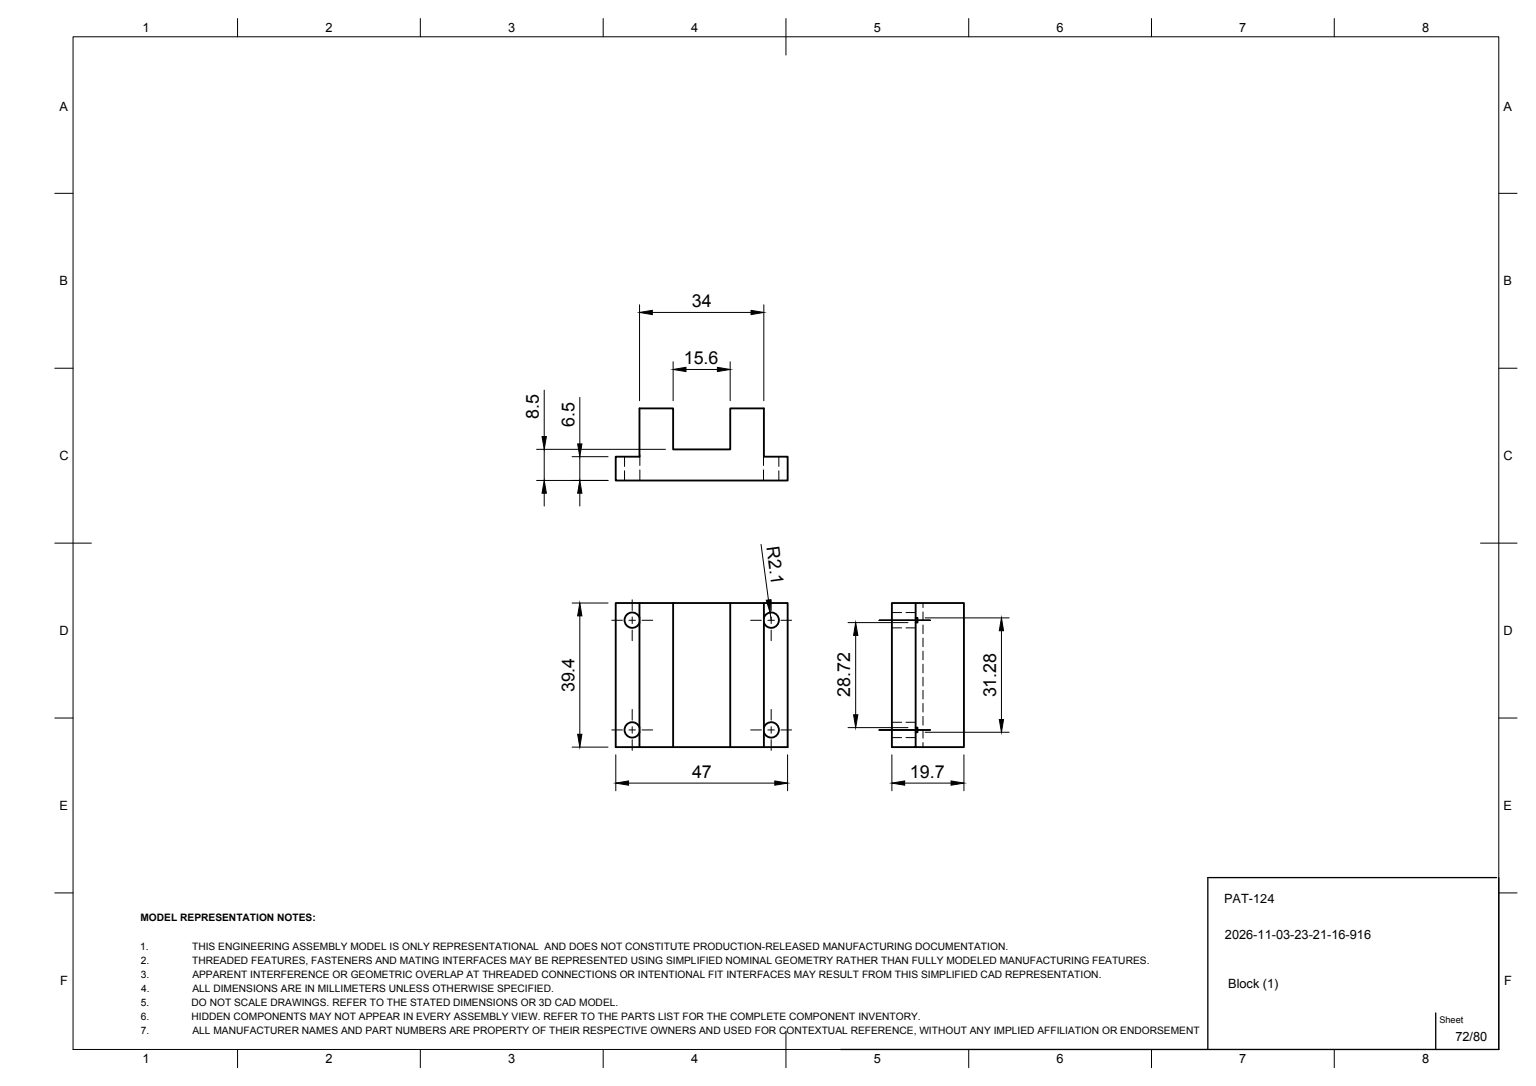
ISO-10303-21;
HEADER;
/* Generated by software containing ST-Developer
 * from STEP Tools, Inc. (www.steptools.com) 
 */

FILE_DESCRIPTION(
/* description */ ('XY cross-slide table'),
/* implementation_level */ '2;1');

FILE_NAME(
/* name */ 'Block (1).step',
/* time_stamp */ '2026-10-28T03:22:46-07:00',
/* author */ (''),
/* organization */ (''),
/* preprocessor_version */ 'ST-DEVELOPER v20.2',
/* originating_system */ 'Autodesk Translation Framework v15.17.0.0',
/* authorisation */ '');

FILE_SCHEMA (('AUTOMOTIVE_DESIGN { 1 0 10303 214 3 1 1 }'));
ENDSEC;

DATA;
#10=MECHANICAL_DESIGN_GEOMETRIC_PRESENTATION_REPRESENTATION('',(#1765),#62984);
#1569=SHAPE_REPRESENTATION_RELATIONSHIP('SRR','None',#63428,#1652);
#1652=ADVANCED_BREP_SHAPE_REPRESENTATION('',(#1873),#62965);
#1765=STYLED_ITEM('',(#63891),#1873);
#1873=MANIFOLD_SOLID_BREP('Body1',#23064);
#2253=FACE_BOUND('',#5529,.T.);
#2254=FACE_BOUND('',#5530,.T.);
#2255=FACE_BOUND('',#5531,.T.);
#2256=FACE_BOUND('',#5532,.T.);
#2731=PLANE('',#25907);
#2732=PLANE('',#25913);
#2733=PLANE('',#25919);
#2734=PLANE('',#25925);
#2735=PLANE('',#25931);
#2736=PLANE('',#25932);
#2737=PLANE('',#25933);
#2738=PLANE('',#25934);
#2739=PLANE('',#25935);
#2740=PLANE('',#25936);
#2741=PLANE('',#25937);
#2742=PLANE('',#25938);
#2743=PLANE('',#25939);
#2744=PLANE('',#25940);
#2745=PLANE('',#25941);
#2746=PLANE('',#25942);
#2747=PLANE('',#25943);
#2748=PLANE('',#25944);
#3835=FACE_OUTER_BOUND('',#5515,.T.);
#3836=FACE_OUTER_BOUND('',#5516,.T.);
#3837=FACE_OUTER_BOUND('',#5517,.T.);
#3838=FACE_OUTER_BOUND('',#5518,.T.);
#3839=FACE_OUTER_BOUND('',#5519,.T.);
#3840=FACE_OUTER_BOUND('',#5520,.T.);
#3841=FACE_OUTER_BOUND('',#5521,.T.);
#3842=FACE_OUTER_BOUND('',#5522,.T.);
#3843=FACE_OUTER_BOUND('',#5523,.T.);
#3844=FACE_OUTER_BOUND('',#5524,.T.);
#3845=FACE_OUTER_BOUND('',#5525,.T.);
#3846=FACE_OUTER_BOUND('',#5526,.T.);
#3847=FACE_OUTER_BOUND('',#5527,.T.);
#3848=FACE_OUTER_BOUND('',#5528,.T.);
#3849=FACE_OUTER_BOUND('',#5533,.T.);
#3850=FACE_OUTER_BOUND('',#5534,.T.);
#3851=FACE_OUTER_BOUND('',#5535,.T.);
#3852=FACE_OUTER_BOUND('',#5536,.T.);
#3853=FACE_OUTER_BOUND('',#5537,.T.);
#3854=FACE_OUTER_BOUND('',#5538,.T.);
#3855=FACE_OUTER_BOUND('',#5539,.T.);
#3856=FACE_OUTER_BOUND('',#5540,.T.);
#5515=EDGE_LOOP('',(#19290,#19291));
#5516=EDGE_LOOP('',(#19292,#19293,#19294,#19295,#19296,#19297,#19298,#19299));
#5517=EDGE_LOOP('',(#19300,#19301));
#5518=EDGE_LOOP('',(#19302,#19303,#19304,#19305,#19306,#19307,#19308,#19309));
#5519=EDGE_LOOP('',(#19310,#19311));
#5520=EDGE_LOOP('',(#19312,#19313,#19314,#19315,#19316,#19317,#19318,#19319));
#5521=EDGE_LOOP('',(#19320,#19321));
#5522=EDGE_LOOP('',(#19322,#19323,#19324,#19325,#19326,#19327,#19328,#19329));
#5523=EDGE_LOOP('',(#19330,#19331,#19332,#19333,#19334,#19335,#19336,#19337,
#19338,#19339,#19340,#19341));
#5524=EDGE_LOOP('',(#19342,#19343,#19344,#19345,#19346,#19347,#19348,#19349,
#19350,#19351,#19352,#19353));
#5525=EDGE_LOOP('',(#19354,#19355,#19356,#19357,#19358,#19359,#19360,#19361,
#19362,#19363,#19364,#19365));
#5526=EDGE_LOOP('',(#19366,#19367,#19368,#19369,#19370,#19371,#19372,#19373,
#19374,#19375));
#5527=EDGE_LOOP('',(#19376,#19377,#19378,#19379));
#5528=EDGE_LOOP('',(#19380,#19381,#19382,#19383));
#5529=EDGE_LOOP('',(#19384));
#5530=EDGE_LOOP('',(#19385));
#5531=EDGE_LOOP('',(#19386));
#5532=EDGE_LOOP('',(#19387));
#5533=EDGE_LOOP('',(#19388,#19389,#19390,#19391));
#5534=EDGE_LOOP('',(#19392,#19393,#19394,#19395,#19396,#19397,#19398,#19399,
#19400,#19401));
#5535=EDGE_LOOP('',(#19402,#19403,#19404,#19405));
#5536=EDGE_LOOP('',(#19406,#19407,#19408,#19409));
#5537=EDGE_LOOP('',(#19410,#19411,#19412,#19413));
#5538=EDGE_LOOP('',(#19414,#19415,#19416,#19417));
#5539=EDGE_LOOP('',(#19418,#19419,#19420,#19421));
#5540=EDGE_LOOP('',(#19422,#19423,#19424,#19425,#19426,#19427,#19428,#19429,
#19430,#19431,#19432,#19433));
#6948=LINE('',#49924,#8435);
#6949=LINE('',#49928,#8436);
#6950=LINE('',#49932,#8437);
#6951=LINE('',#49936,#8438);
#6952=LINE('',#49940,#8439);
#6953=LINE('',#49944,#8440);
#6954=LINE('',#49948,#8441);
#6955=LINE('',#49952,#8442);
#6956=LINE('',#49956,#8443);
#6957=LINE('',#49960,#8444);
#6958=LINE('',#49964,#8445);
#6959=LINE('',#49968,#8446);
#6960=LINE('',#49972,#8447);
#6961=LINE('',#49976,#8448);
#6962=LINE('',#49980,#8449);
#6963=LINE('',#49984,#8450);
#6964=LINE('',#49986,#8451);
#6965=LINE('',#49988,#8452);
#6966=LINE('',#49990,#8453);
#6967=LINE('',#49992,#8454);
#6968=LINE('',#49994,#8455);
#6969=LINE('',#49995,#8456);
#6970=LINE('',#49997,#8457);
#6971=LINE('',#49999,#8458);
#6972=LINE('',#50001,#8459);
#6973=LINE('',#50003,#8460);
#6974=LINE('',#50005,#8461);
#6975=LINE('',#50006,#8462);
#6976=LINE('',#50009,#8463);
#6977=LINE('',#50011,#8464);
#6978=LINE('',#50013,#8465);
#6979=LINE('',#50015,#8466);
#6980=LINE('',#50016,#8467);
#6981=LINE('',#50018,#8468);
#6982=LINE('',#50020,#8469);
#6983=LINE('',#50022,#8470);
#6984=LINE('',#50024,#8471);
#6985=LINE('',#50025,#8472);
#6986=LINE('',#50028,#8473);
#6987=LINE('',#50029,#8474);
#6988=LINE('',#50032,#8475);
#6989=LINE('',#50033,#8476);
#6990=LINE('',#50036,#8477);
#6991=LINE('',#50037,#8478);
#6992=LINE('',#50040,#8479);
#6993=LINE('',#50041,#8480);
#6994=LINE('',#50043,#8481);
#6995=LINE('',#50046,#8482);
#6996=LINE('',#50047,#8483);
#6997=LINE('',#50050,#8484);
#6998=LINE('',#50051,#8485);
#6999=LINE('',#50054,#8486);
#7000=LINE('',#50055,#8487);
#7001=LINE('',#50058,#8488);
#7002=LINE('',#50059,#8489);
#7003=LINE('',#50061,#8490);
#8435=VECTOR('',#31319,1.);
#8436=VECTOR('',#31324,1.);
#8437=VECTOR('',#31327,0.21);
#8438=VECTOR('',#31332,1.);
#8439=VECTOR('',#31335,1.);
#8440=VECTOR('',#31340,1.);
#8441=VECTOR('',#31343,0.21);
#8442=VECTOR('',#31348,1.);
#8443=VECTOR('',#31351,1.);
#8444=VECTOR('',#31356,1.);
#8445=VECTOR('',#31359,0.21);
#8446=VECTOR('',#31364,1.);
#8447=VECTOR('',#31367,1.);
#8448=VECTOR('',#31372,1.);
#8449=VECTOR('',#31375,0.21);
#8450=VECTOR('',#31380,1.);
#8451=VECTOR('',#31383,1.);
#8452=VECTOR('',#31384,1.);
#8453=VECTOR('',#31385,1.);
#8454=VECTOR('',#31386,1.);
#8455=VECTOR('',#31387,1.);
#8456=VECTOR('',#31388,1.);
#8457=VECTOR('',#31391,1.);
#8458=VECTOR('',#31392,1.);
#8459=VECTOR('',#31393,1.);
#8460=VECTOR('',#31394,1.);
#8461=VECTOR('',#31395,1.);
#8462=VECTOR('',#31396,1.);
#8463=VECTOR('',#31399,1.);
#8464=VECTOR('',#31400,1.);
#8465=VECTOR('',#31401,1.);
#8466=VECTOR('',#31402,1.);
#8467=VECTOR('',#31403,1.);
#8468=VECTOR('',#31404,1.);
#8469=VECTOR('',#31405,1.);
#8470=VECTOR('',#31406,1.);
#8471=VECTOR('',#31407,1.);
#8472=VECTOR('',#31408,1.);
#8473=VECTOR('',#31411,1.);
#8474=VECTOR('',#31412,1.);
#8475=VECTOR('',#31415,1.);
#8476=VECTOR('',#31416,1.);
#8477=VECTOR('',#31419,1.);
#8478=VECTOR('',#31420,1.);
#8479=VECTOR('',#31423,1.);
#8480=VECTOR('',#31424,1.);
#8481=VECTOR('',#31427,1.);
#8482=VECTOR('',#31430,1.);
#8483=VECTOR('',#31431,1.);
#8484=VECTOR('',#31434,1.);
#8485=VECTOR('',#31435,1.);
#8486=VECTOR('',#31438,1.);
#8487=VECTOR('',#31439,1.);
#8488=VECTOR('',#31442,1.);
#8489=VECTOR('',#31443,1.);
#8490=VECTOR('',#31446,1.);
#9655=CIRCLE('',#25908,0.21);
#9656=CIRCLE('',#25910,0.21);
#9657=CIRCLE('',#25911,0.21);
#9658=CIRCLE('',#25912,0.21);
#9659=CIRCLE('',#25914,0.21);
#9660=CIRCLE('',#25916,0.21);
#9661=CIRCLE('',#25917,0.21);
#9662=CIRCLE('',#25918,0.21);
#9663=CIRCLE('',#25920,0.21);
#9664=CIRCLE('',#25922,0.21);
#9665=CIRCLE('',#25923,0.21);
#9666=CIRCLE('',#25924,0.21);
#9667=CIRCLE('',#25926,0.21);
#9668=CIRCLE('',#25928,0.21);
#9669=CIRCLE('',#25929,0.21);
#9670=CIRCLE('',#25930,0.21);
#11258=VERTEX_POINT('',#49922);
#11259=VERTEX_POINT('',#49923);
#11260=VERTEX_POINT('',#49927);
#11261=VERTEX_POINT('',#49929);
#11262=VERTEX_POINT('',#49931);
#11263=VERTEX_POINT('',#49934);
#11264=VERTEX_POINT('',#49938);
#11265=VERTEX_POINT('',#49939);
#11266=VERTEX_POINT('',#49943);
#11267=VERTEX_POINT('',#49945);
#11268=VERTEX_POINT('',#49947);
#11269=VERTEX_POINT('',#49950);
#11270=VERTEX_POINT('',#49954);
#11271=VERTEX_POINT('',#49955);
#11272=VERTEX_POINT('',#49959);
#11273=VERTEX_POINT('',#49961);
#11274=VERTEX_POINT('',#49963);
#11275=VERTEX_POINT('',#49966);
#11276=VERTEX_POINT('',#49970);
#11277=VERTEX_POINT('',#49971);
#11278=VERTEX_POINT('',#49975);
#11279=VERTEX_POINT('',#49977);
#11280=VERTEX_POINT('',#49979);
#11281=VERTEX_POINT('',#49982);
#11282=VERTEX_POINT('',#49987);
#11283=VERTEX_POINT('',#49989);
#11284=VERTEX_POINT('',#49991);
#11285=VERTEX_POINT('',#49993);
#11286=VERTEX_POINT('',#49998);
#11287=VERTEX_POINT('',#50000);
#11288=VERTEX_POINT('',#50002);
#11289=VERTEX_POINT('',#50004);
#11290=VERTEX_POINT('',#50008);
#11291=VERTEX_POINT('',#50010);
#11292=VERTEX_POINT('',#50012);
#11293=VERTEX_POINT('',#50014);
#11294=VERTEX_POINT('',#50017);
#11295=VERTEX_POINT('',#50019);
#11296=VERTEX_POINT('',#50021);
#11297=VERTEX_POINT('',#50023);
#11298=VERTEX_POINT('',#50027);
#11299=VERTEX_POINT('',#50031);
#11300=VERTEX_POINT('',#50035);
#11301=VERTEX_POINT('',#50039);
#11302=VERTEX_POINT('',#50045);
#11303=VERTEX_POINT('',#50049);
#11304=VERTEX_POINT('',#50053);
#11305=VERTEX_POINT('',#50057);
#14029=EDGE_CURVE('',#11258,#11259,#6948,.T.);
#14030=EDGE_CURVE('',#11258,#11259,#9655,.T.);
#14031=EDGE_CURVE('',#11260,#11258,#6949,.T.);
#14032=EDGE_CURVE('',#11261,#11260,#9656,.T.);
#14033=EDGE_CURVE('',#11261,#11262,#6950,.T.);
#14034=EDGE_CURVE('',#11262,#11262,#9657,.T.);
#14035=EDGE_CURVE('',#11263,#11261,#9658,.T.);
#14036=EDGE_CURVE('',#11259,#11263,#6951,.T.);
#14037=EDGE_CURVE('',#11264,#11265,#6952,.T.);
#14038=EDGE_CURVE('',#11264,#11265,#9659,.T.);
#14039=EDGE_CURVE('',#11266,#11264,#6953,.T.);
#14040=EDGE_CURVE('',#11267,#11266,#9660,.T.);
#14041=EDGE_CURVE('',#11267,#11268,#6954,.T.);
#14042=EDGE_CURVE('',#11268,#11268,#9661,.T.);
#14043=EDGE_CURVE('',#11269,#11267,#9662,.T.);
#14044=EDGE_CURVE('',#11265,#11269,#6955,.T.);
#14045=EDGE_CURVE('',#11270,#11271,#6956,.T.);
#14046=EDGE_CURVE('',#11270,#11271,#9663,.T.);
#14047=EDGE_CURVE('',#11272,#11270,#6957,.T.);
#14048=EDGE_CURVE('',#11273,#11272,#9664,.T.);
#14049=EDGE_CURVE('',#11273,#11274,#6958,.T.);
#14050=EDGE_CURVE('',#11274,#11274,#9665,.T.);
#14051=EDGE_CURVE('',#11275,#11273,#9666,.T.);
#14052=EDGE_CURVE('',#11271,#11275,#6959,.T.);
#14053=EDGE_CURVE('',#11276,#11277,#6960,.T.);
#14054=EDGE_CURVE('',#11276,#11277,#9667,.T.);
#14055=EDGE_CURVE('',#11278,#11276,#6961,.T.);
#14056=EDGE_CURVE('',#11279,#11278,#9668,.T.);
#14057=EDGE_CURVE('',#11279,#11280,#6962,.T.);
#14058=EDGE_CURVE('',#11280,#11280,#9669,.T.);
#14059=EDGE_CURVE('',#11281,#11279,#9670,.T.);
#14060=EDGE_CURVE('',#11277,#11281,#6963,.T.);
#14061=EDGE_CURVE('',#11263,#11272,#6964,.T.);
#14062=EDGE_CURVE('',#11275,#11282,#6965,.T.);
#14063=EDGE_CURVE('',#11283,#11282,#6966,.T.);
#14064=EDGE_CURVE('',#11283,#11284,#6967,.T.);
#14065=EDGE_CURVE('',#11285,#11284,#6968,.T.);
#14066=EDGE_CURVE('',#11285,#11260,#6969,.T.);
#14067=EDGE_CURVE('',#11269,#11278,#6970,.T.);
#14068=EDGE_CURVE('',#11281,#11286,#6971,.T.);
#14069=EDGE_CURVE('',#11287,#11286,#6972,.T.);
#14070=EDGE_CURVE('',#11288,#11287,#6973,.T.);
#14071=EDGE_CURVE('',#11289,#11288,#6974,.T.);
#14072=EDGE_CURVE('',#11289,#11266,#6975,.T.);
#14073=EDGE_CURVE('',#11282,#11290,#6976,.T.);
#14074=EDGE_CURVE('',#11290,#11291,#6977,.T.);
#14075=EDGE_CURVE('',#11291,#11292,#6978,.T.);
#14076=EDGE_CURVE('',#11292,#11293,#6979,.T.);
#14077=EDGE_CURVE('',#11293,#11289,#6980,.T.);
#14078=EDGE_CURVE('',#11288,#11294,#6981,.T.);
#14079=EDGE_CURVE('',#11294,#11295,#6982,.T.);
#14080=EDGE_CURVE('',#11295,#11296,#6983,.T.);
#14081=EDGE_CURVE('',#11296,#11297,#6984,.T.);
#14082=EDGE_CURVE('',#11297,#11283,#6985,.T.);
#14083=EDGE_CURVE('',#11298,#11285,#6986,.T.);
#14084=EDGE_CURVE('',#11290,#11298,#6987,.T.);
#14085=EDGE_CURVE('',#11299,#11298,#6988,.T.);
#14086=EDGE_CURVE('',#11291,#11299,#6989,.T.);
#14087=EDGE_CURVE('',#11300,#11299,#6990,.T.);
#14088=EDGE_CURVE('',#11292,#11300,#6991,.T.);
#14089=EDGE_CURVE('',#11301,#11300,#6992,.T.);
#14090=EDGE_CURVE('',#11293,#11301,#6993,.T.);
#14091=EDGE_CURVE('',#11286,#11301,#6994,.T.);
#14092=EDGE_CURVE('',#11302,#11287,#6995,.T.);
#14093=EDGE_CURVE('',#11294,#11302,#6996,.T.);
#14094=EDGE_CURVE('',#11303,#11302,#6997,.T.);
#14095=EDGE_CURVE('',#11295,#11303,#6998,.T.);
#14096=EDGE_CURVE('',#11304,#11303,#6999,.T.);
#14097=EDGE_CURVE('',#11296,#11304,#7000,.T.);
#14098=EDGE_CURVE('',#11305,#11304,#7001,.T.);
#14099=EDGE_CURVE('',#11297,#11305,#7002,.T.);
#14100=EDGE_CURVE('',#11284,#11305,#7003,.T.);
#19290=ORIENTED_EDGE('',*,*,#14029,.F.);
#19291=ORIENTED_EDGE('',*,*,#14030,.T.);
#19292=ORIENTED_EDGE('',*,*,#14031,.F.);
#19293=ORIENTED_EDGE('',*,*,#14032,.F.);
#19294=ORIENTED_EDGE('',*,*,#14033,.T.);
#19295=ORIENTED_EDGE('',*,*,#14034,.F.);
#19296=ORIENTED_EDGE('',*,*,#14033,.F.);
#19297=ORIENTED_EDGE('',*,*,#14035,.F.);
#19298=ORIENTED_EDGE('',*,*,#14036,.F.);
#19299=ORIENTED_EDGE('',*,*,#14030,.F.);
#19300=ORIENTED_EDGE('',*,*,#14037,.F.);
#19301=ORIENTED_EDGE('',*,*,#14038,.T.);
#19302=ORIENTED_EDGE('',*,*,#14039,.F.);
#19303=ORIENTED_EDGE('',*,*,#14040,.F.);
#19304=ORIENTED_EDGE('',*,*,#14041,.T.);
#19305=ORIENTED_EDGE('',*,*,#14042,.F.);
#19306=ORIENTED_EDGE('',*,*,#14041,.F.);
#19307=ORIENTED_EDGE('',*,*,#14043,.F.);
#19308=ORIENTED_EDGE('',*,*,#14044,.F.);
#19309=ORIENTED_EDGE('',*,*,#14038,.F.);
#19310=ORIENTED_EDGE('',*,*,#14045,.F.);
#19311=ORIENTED_EDGE('',*,*,#14046,.T.);
#19312=ORIENTED_EDGE('',*,*,#14047,.F.);
#19313=ORIENTED_EDGE('',*,*,#14048,.F.);
#19314=ORIENTED_EDGE('',*,*,#14049,.T.);
#19315=ORIENTED_EDGE('',*,*,#14050,.F.);
#19316=ORIENTED_EDGE('',*,*,#14049,.F.);
#19317=ORIENTED_EDGE('',*,*,#14051,.F.);
#19318=ORIENTED_EDGE('',*,*,#14052,.F.);
#19319=ORIENTED_EDGE('',*,*,#14046,.F.);
#19320=ORIENTED_EDGE('',*,*,#14053,.F.);
#19321=ORIENTED_EDGE('',*,*,#14054,.T.);
#19322=ORIENTED_EDGE('',*,*,#14055,.F.);
#19323=ORIENTED_EDGE('',*,*,#14056,.F.);
#19324=ORIENTED_EDGE('',*,*,#14057,.T.);
#19325=ORIENTED_EDGE('',*,*,#14058,.F.);
#19326=ORIENTED_EDGE('',*,*,#14057,.F.);
#19327=ORIENTED_EDGE('',*,*,#14059,.F.);
#19328=ORIENTED_EDGE('',*,*,#14060,.F.);
#19329=ORIENTED_EDGE('',*,*,#14054,.F.);
#19330=ORIENTED_EDGE('',*,*,#14031,.T.);
#19331=ORIENTED_EDGE('',*,*,#14029,.T.);
#19332=ORIENTED_EDGE('',*,*,#14036,.T.);
#19333=ORIENTED_EDGE('',*,*,#14061,.T.);
#19334=ORIENTED_EDGE('',*,*,#14047,.T.);
#19335=ORIENTED_EDGE('',*,*,#14045,.T.);
#19336=ORIENTED_EDGE('',*,*,#14052,.T.);
#19337=ORIENTED_EDGE('',*,*,#14062,.T.);
#19338=ORIENTED_EDGE('',*,*,#14063,.F.);
#19339=ORIENTED_EDGE('',*,*,#14064,.T.);
#19340=ORIENTED_EDGE('',*,*,#14065,.F.);
#19341=ORIENTED_EDGE('',*,*,#14066,.T.);
#19342=ORIENTED_EDGE('',*,*,#14039,.T.);
#19343=ORIENTED_EDGE('',*,*,#14037,.T.);
#19344=ORIENTED_EDGE('',*,*,#14044,.T.);
#19345=ORIENTED_EDGE('',*,*,#14067,.T.);
#19346=ORIENTED_EDGE('',*,*,#14055,.T.);
#19347=ORIENTED_EDGE('',*,*,#14053,.T.);
#19348=ORIENTED_EDGE('',*,*,#14060,.T.);
#19349=ORIENTED_EDGE('',*,*,#14068,.T.);
#19350=ORIENTED_EDGE('',*,*,#14069,.F.);
#19351=ORIENTED_EDGE('',*,*,#14070,.F.);
#19352=ORIENTED_EDGE('',*,*,#14071,.F.);
#19353=ORIENTED_EDGE('',*,*,#14072,.T.);
#19354=ORIENTED_EDGE('',*,*,#14063,.T.);
#19355=ORIENTED_EDGE('',*,*,#14073,.T.);
#19356=ORIENTED_EDGE('',*,*,#14074,.T.);
#19357=ORIENTED_EDGE('',*,*,#14075,.T.);
#19358=ORIENTED_EDGE('',*,*,#14076,.T.);
#19359=ORIENTED_EDGE('',*,*,#14077,.T.);
#19360=ORIENTED_EDGE('',*,*,#14071,.T.);
#19361=ORIENTED_EDGE('',*,*,#14078,.T.);
#19362=ORIENTED_EDGE('',*,*,#14079,.T.);
#19363=ORIENTED_EDGE('',*,*,#14080,.T.);
#19364=ORIENTED_EDGE('',*,*,#14081,.T.);
#19365=ORIENTED_EDGE('',*,*,#14082,.T.);
#19366=ORIENTED_EDGE('',*,*,#14035,.T.);
#19367=ORIENTED_EDGE('',*,*,#14032,.T.);
#19368=ORIENTED_EDGE('',*,*,#14066,.F.);
#19369=ORIENTED_EDGE('',*,*,#14083,.F.);
#19370=ORIENTED_EDGE('',*,*,#14084,.F.);
#19371=ORIENTED_EDGE('',*,*,#14073,.F.);
#19372=ORIENTED_EDGE('',*,*,#14062,.F.);
#19373=ORIENTED_EDGE('',*,*,#14051,.T.);
#19374=ORIENTED_EDGE('',*,*,#14048,.T.);
#19375=ORIENTED_EDGE('',*,*,#14061,.F.);
#19376=ORIENTED_EDGE('',*,*,#14084,.T.);
#19377=ORIENTED_EDGE('',*,*,#14085,.F.);
#19378=ORIENTED_EDGE('',*,*,#14086,.F.);
#19379=ORIENTED_EDGE('',*,*,#14074,.F.);
#19380=ORIENTED_EDGE('',*,*,#14086,.T.);
#19381=ORIENTED_EDGE('',*,*,#14087,.F.);
#19382=ORIENTED_EDGE('',*,*,#14088,.F.);
#19383=ORIENTED_EDGE('',*,*,#14075,.F.);
#19384=ORIENTED_EDGE('',*,*,#14034,.T.);
#19385=ORIENTED_EDGE('',*,*,#14042,.T.);
#19386=ORIENTED_EDGE('',*,*,#14050,.T.);
#19387=ORIENTED_EDGE('',*,*,#14058,.T.);
#19388=ORIENTED_EDGE('',*,*,#14088,.T.);
#19389=ORIENTED_EDGE('',*,*,#14089,.F.);
#19390=ORIENTED_EDGE('',*,*,#14090,.F.);
#19391=ORIENTED_EDGE('',*,*,#14076,.F.);
#19392=ORIENTED_EDGE('',*,*,#14043,.T.);
#19393=ORIENTED_EDGE('',*,*,#14040,.T.);
#19394=ORIENTED_EDGE('',*,*,#14072,.F.);
#19395=ORIENTED_EDGE('',*,*,#14077,.F.);
#19396=ORIENTED_EDGE('',*,*,#14090,.T.);
#19397=ORIENTED_EDGE('',*,*,#14091,.F.);
#19398=ORIENTED_EDGE('',*,*,#14068,.F.);
#19399=ORIENTED_EDGE('',*,*,#14059,.T.);
#19400=ORIENTED_EDGE('',*,*,#14056,.T.);
#19401=ORIENTED_EDGE('',*,*,#14067,.F.);
#19402=ORIENTED_EDGE('',*,*,#14070,.T.);
#19403=ORIENTED_EDGE('',*,*,#14092,.F.);
#19404=ORIENTED_EDGE('',*,*,#14093,.F.);
#19405=ORIENTED_EDGE('',*,*,#14078,.F.);
#19406=ORIENTED_EDGE('',*,*,#14093,.T.);
#19407=ORIENTED_EDGE('',*,*,#14094,.F.);
#19408=ORIENTED_EDGE('',*,*,#14095,.F.);
#19409=ORIENTED_EDGE('',*,*,#14079,.F.);
#19410=ORIENTED_EDGE('',*,*,#14095,.T.);
#19411=ORIENTED_EDGE('',*,*,#14096,.F.);
#19412=ORIENTED_EDGE('',*,*,#14097,.F.);
#19413=ORIENTED_EDGE('',*,*,#14080,.F.);
#19414=ORIENTED_EDGE('',*,*,#14097,.T.);
#19415=ORIENTED_EDGE('',*,*,#14098,.F.);
#19416=ORIENTED_EDGE('',*,*,#14099,.F.);
#19417=ORIENTED_EDGE('',*,*,#14081,.F.);
#19418=ORIENTED_EDGE('',*,*,#14099,.T.);
#19419=ORIENTED_EDGE('',*,*,#14100,.F.);
#19420=ORIENTED_EDGE('',*,*,#14064,.F.);
#19421=ORIENTED_EDGE('',*,*,#14082,.F.);
#19422=ORIENTED_EDGE('',*,*,#14065,.T.);
#19423=ORIENTED_EDGE('',*,*,#14100,.T.);
#19424=ORIENTED_EDGE('',*,*,#14098,.T.);
#19425=ORIENTED_EDGE('',*,*,#14096,.T.);
#19426=ORIENTED_EDGE('',*,*,#14094,.T.);
#19427=ORIENTED_EDGE('',*,*,#14092,.T.);
#19428=ORIENTED_EDGE('',*,*,#14069,.T.);
#19429=ORIENTED_EDGE('',*,*,#14091,.T.);
#19430=ORIENTED_EDGE('',*,*,#14089,.T.);
#19431=ORIENTED_EDGE('',*,*,#14087,.T.);
#19432=ORIENTED_EDGE('',*,*,#14085,.T.);
#19433=ORIENTED_EDGE('',*,*,#14083,.T.);
#21462=CYLINDRICAL_SURFACE('',#25909,0.21);
#21463=CYLINDRICAL_SURFACE('',#25915,0.21);
#21464=CYLINDRICAL_SURFACE('',#25921,0.21);
#21465=CYLINDRICAL_SURFACE('',#25927,0.21);
#22616=ADVANCED_FACE('',(#3835),#2731,.T.);
#22617=ADVANCED_FACE('',(#3836),#21462,.F.);
#22618=ADVANCED_FACE('',(#3837),#2732,.T.);
#22619=ADVANCED_FACE('',(#3838),#21463,.F.);
#22620=ADVANCED_FACE('',(#3839),#2733,.T.);
#22621=ADVANCED_FACE('',(#3840),#21464,.F.);
#22622=ADVANCED_FACE('',(#3841),#2734,.T.);
#22623=ADVANCED_FACE('',(#3842),#21465,.F.);
#22624=ADVANCED_FACE('',(#3843),#2735,.T.);
#22625=ADVANCED_FACE('',(#3844),#2736,.T.);
#22626=ADVANCED_FACE('',(#3845),#2737,.T.);
#22627=ADVANCED_FACE('',(#3846),#2738,.T.);
#22628=ADVANCED_FACE('',(#3847),#2739,.T.);
#22629=ADVANCED_FACE('',(#3848,#2253,#2254,#2255,#2256),#2740,.T.);
#22630=ADVANCED_FACE('',(#3849),#2741,.T.);
#22631=ADVANCED_FACE('',(#3850),#2742,.T.);
#22632=ADVANCED_FACE('',(#3851),#2743,.T.);
#22633=ADVANCED_FACE('',(#3852),#2744,.T.);
#22634=ADVANCED_FACE('',(#3853),#2745,.T.);
#22635=ADVANCED_FACE('',(#3854),#2746,.T.);
#22636=ADVANCED_FACE('',(#3855),#2747,.T.);
#22637=ADVANCED_FACE('',(#3856),#2748,.T.);
#23064=CLOSED_SHELL('',(#22616,#22617,#22618,#22619,#22620,#22621,#22622,
#22623,#22624,#22625,#22626,#22627,#22628,#22629,#22630,#22631,#22632,#22633,
#22634,#22635,#22636,#22637));
#25906=AXIS2_PLACEMENT_3D('',#49920,#31315,#31316);
#25907=AXIS2_PLACEMENT_3D('',#49921,#31317,#31318);
#25908=AXIS2_PLACEMENT_3D('',#49925,#31320,#31321);
#25909=AXIS2_PLACEMENT_3D('',#49926,#31322,#31323);
#25910=AXIS2_PLACEMENT_3D('',#49930,#31325,#31326);
#25911=AXIS2_PLACEMENT_3D('',#49933,#31328,#31329);
#25912=AXIS2_PLACEMENT_3D('',#49935,#31330,#31331);
#25913=AXIS2_PLACEMENT_3D('',#49937,#31333,#31334);
#25914=AXIS2_PLACEMENT_3D('',#49941,#31336,#31337);
#25915=AXIS2_PLACEMENT_3D('',#49942,#31338,#31339);
#25916=AXIS2_PLACEMENT_3D('',#49946,#31341,#31342);
#25917=AXIS2_PLACEMENT_3D('',#49949,#31344,#31345);
#25918=AXIS2_PLACEMENT_3D('',#49951,#31346,#31347);
#25919=AXIS2_PLACEMENT_3D('',#49953,#31349,#31350);
#25920=AXIS2_PLACEMENT_3D('',#49957,#31352,#31353);
#25921=AXIS2_PLACEMENT_3D('',#49958,#31354,#31355);
#25922=AXIS2_PLACEMENT_3D('',#49962,#31357,#31358);
#25923=AXIS2_PLACEMENT_3D('',#49965,#31360,#31361);
#25924=AXIS2_PLACEMENT_3D('',#49967,#31362,#31363);
#25925=AXIS2_PLACEMENT_3D('',#49969,#31365,#31366);
#25926=AXIS2_PLACEMENT_3D('',#49973,#31368,#31369);
#25927=AXIS2_PLACEMENT_3D('',#49974,#31370,#31371);
#25928=AXIS2_PLACEMENT_3D('',#49978,#31373,#31374);
#25929=AXIS2_PLACEMENT_3D('',#49981,#31376,#31377);
#25930=AXIS2_PLACEMENT_3D('',#49983,#31378,#31379);
#25931=AXIS2_PLACEMENT_3D('',#49985,#31381,#31382);
#25932=AXIS2_PLACEMENT_3D('',#49996,#31389,#31390);
#25933=AXIS2_PLACEMENT_3D('',#50007,#31397,#31398);
#25934=AXIS2_PLACEMENT_3D('',#50026,#31409,#31410);
#25935=AXIS2_PLACEMENT_3D('',#50030,#31413,#31414);
#25936=AXIS2_PLACEMENT_3D('',#50034,#31417,#31418);
#25937=AXIS2_PLACEMENT_3D('',#50038,#31421,#31422);
#25938=AXIS2_PLACEMENT_3D('',#50042,#31425,#31426);
#25939=AXIS2_PLACEMENT_3D('',#50044,#31428,#31429);
#25940=AXIS2_PLACEMENT_3D('',#50048,#31432,#31433);
#25941=AXIS2_PLACEMENT_3D('',#50052,#31436,#31437);
#25942=AXIS2_PLACEMENT_3D('',#50056,#31440,#31441);
#25943=AXIS2_PLACEMENT_3D('',#50060,#31444,#31445);
#25944=AXIS2_PLACEMENT_3D('',#50062,#31447,#31448);
#31315=DIRECTION('axis',(0.,0.,1.));
#31316=DIRECTION('refdir',(1.,0.,0.));
#31317=DIRECTION('center_axis',(0.,0.,1.));
#31318=DIRECTION('ref_axis',(1.,0.,0.));
#31319=DIRECTION('',(-1.,0.,0.));
#31320=DIRECTION('center_axis',(0.,0.,1.));
#31321=DIRECTION('ref_axis',(1.,0.,0.));
#31322=DIRECTION('center_axis',(0.,0.,1.));
#31323=DIRECTION('ref_axis',(1.,0.,0.));
#31324=DIRECTION('',(0.,0.,-1.));
#31325=DIRECTION('center_axis',(0.,0.,1.));
#31326=DIRECTION('ref_axis',(1.,0.,0.));
#31327=DIRECTION('',(0.,0.,1.));
#31328=DIRECTION('center_axis',(0.,0.,-1.));
#31329=DIRECTION('ref_axis',(1.,0.,0.));
#31330=DIRECTION('center_axis',(0.,0.,1.));
#31331=DIRECTION('ref_axis',(1.,0.,0.));
#31332=DIRECTION('',(0.,0.,1.));
#31333=DIRECTION('center_axis',(0.,0.,1.));
#31334=DIRECTION('ref_axis',(1.,0.,0.));
#31335=DIRECTION('',(1.,0.,0.));
#31336=DIRECTION('center_axis',(0.,0.,1.));
#31337=DIRECTION('ref_axis',(1.,0.,0.));
#31338=DIRECTION('center_axis',(0.,0.,1.));
#31339=DIRECTION('ref_axis',(1.,0.,0.));
#31340=DIRECTION('',(0.,0.,-1.));
#31341=DIRECTION('center_axis',(0.,0.,1.));
#31342=DIRECTION('ref_axis',(1.,0.,0.));
#31343=DIRECTION('',(0.,0.,1.));
#31344=DIRECTION('center_axis',(0.,0.,-1.));
#31345=DIRECTION('ref_axis',(1.,0.,0.));
#31346=DIRECTION('center_axis',(0.,0.,1.));
#31347=DIRECTION('ref_axis',(1.,0.,0.));
#31348=DIRECTION('',(0.,0.,1.));
#31349=DIRECTION('center_axis',(0.,0.,1.));
#31350=DIRECTION('ref_axis',(1.,0.,0.));
#31351=DIRECTION('',(-1.,0.,0.));
#31352=DIRECTION('center_axis',(0.,0.,1.));
#31353=DIRECTION('ref_axis',(1.,0.,0.));
#31354=DIRECTION('center_axis',(0.,0.,1.));
#31355=DIRECTION('ref_axis',(1.,0.,0.));
#31356=DIRECTION('',(0.,0.,-1.));
#31357=DIRECTION('center_axis',(0.,0.,1.));
#31358=DIRECTION('ref_axis',(1.,0.,0.));
#31359=DIRECTION('',(0.,0.,1.));
#31360=DIRECTION('center_axis',(0.,0.,-1.));
#31361=DIRECTION('ref_axis',(1.,0.,0.));
#31362=DIRECTION('center_axis',(0.,0.,1.));
#31363=DIRECTION('ref_axis',(1.,0.,0.));
#31364=DIRECTION('',(0.,0.,1.));
#31365=DIRECTION('center_axis',(0.,0.,1.));
#31366=DIRECTION('ref_axis',(1.,0.,0.));
#31367=DIRECTION('',(1.,0.,0.));
#31368=DIRECTION('center_axis',(0.,0.,1.));
#31369=DIRECTION('ref_axis',(1.,0.,0.));
#31370=DIRECTION('center_axis',(0.,0.,1.));
#31371=DIRECTION('ref_axis',(1.,0.,0.));
#31372=DIRECTION('',(0.,0.,-1.));
#31373=DIRECTION('center_axis',(0.,0.,1.));
#31374=DIRECTION('ref_axis',(1.,0.,0.));
#31375=DIRECTION('',(0.,0.,1.));
#31376=DIRECTION('center_axis',(0.,0.,-1.));
#31377=DIRECTION('ref_axis',(1.,0.,0.));
#31378=DIRECTION('center_axis',(0.,0.,1.));
#31379=DIRECTION('ref_axis',(1.,0.,0.));
#31380=DIRECTION('',(0.,0.,1.));
#31381=DIRECTION('center_axis',(0.,-1.,0.));
#31382=DIRECTION('ref_axis',(0.,0.,-1.));
#31383=DIRECTION('',(-1.,0.,0.));
#31384=DIRECTION('',(-1.,0.,0.));
#31385=DIRECTION('',(0.,0.,1.));
#31386=DIRECTION('',(1.,0.,0.));
#31387=DIRECTION('',(0.,0.,-1.));
#31388=DIRECTION('',(-1.,0.,0.));
#31389=DIRECTION('center_axis',(0.,1.,0.));
#31390=DIRECTION('ref_axis',(0.,0.,1.));
#31391=DIRECTION('',(1.,0.,0.));
#31392=DIRECTION('',(1.,0.,0.));
#31393=DIRECTION('',(0.,0.,1.));
#31394=DIRECTION('',(1.,0.,0.));
#31395=DIRECTION('',(0.,0.,-1.));
#31396=DIRECTION('',(1.,0.,0.));
#31397=DIRECTION('center_axis',(-1.,0.,0.));
#31398=DIRECTION('ref_axis',(0.,0.,1.));
#31399=DIRECTION('',(0.,-1.,0.));
#31400=DIRECTION('',(0.,0.,1.));
#31401=DIRECTION('',(0.,1.,0.));
#31402=DIRECTION('',(0.,0.,-1.));
#31403=DIRECTION('',(0.,-1.,0.));
#31404=DIRECTION('',(0.,-1.,0.));
#31405=DIRECTION('',(0.,0.,1.));
#31406=DIRECTION('',(0.,-1.,0.));
#31407=DIRECTION('',(0.,0.,-1.));
#31408=DIRECTION('',(0.,-1.,0.));
#31409=DIRECTION('center_axis',(0.,0.,-1.));
#31410=DIRECTION('ref_axis',(0.,1.,0.));
#31411=DIRECTION('',(0.,1.,0.));
#31412=DIRECTION('',(1.,0.,0.));
#31413=DIRECTION('center_axis',(0.,-1.,0.));
#31414=DIRECTION('ref_axis',(0.,0.,-1.));
#31415=DIRECTION('',(0.,0.,-1.));
#31416=DIRECTION('',(1.,0.,0.));
#31417=DIRECTION('center_axis',(0.,0.,1.));
#31418=DIRECTION('ref_axis',(0.,-1.,0.));
#31419=DIRECTION('',(0.,-1.,0.));
#31420=DIRECTION('',(1.,0.,0.));
#31421=DIRECTION('center_axis',(0.,1.,0.));
#31422=DIRECTION('ref_axis',(0.,0.,1.));
#31423=DIRECTION('',(0.,0.,1.));
#31424=DIRECTION('',(1.,0.,0.));
#31425=DIRECTION('center_axis',(0.,0.,-1.));
#31426=DIRECTION('ref_axis',(0.,1.,0.));
#31427=DIRECTION('',(0.,1.,0.));
#31428=DIRECTION('center_axis',(0.,0.,-1.));
#31429=DIRECTION('ref_axis',(0.,1.,0.));
#31430=DIRECTION('',(0.,1.,0.));
#31431=DIRECTION('',(1.,0.,0.));
#31432=DIRECTION('center_axis',(0.,-1.,0.));
#31433=DIRECTION('ref_axis',(0.,0.,-1.));
#31434=DIRECTION('',(0.,0.,-1.));
#31435=DIRECTION('',(1.,0.,0.));
#31436=DIRECTION('center_axis',(0.,0.,-1.));
#31437=DIRECTION('ref_axis',(0.,1.,0.));
#31438=DIRECTION('',(0.,1.,0.));
#31439=DIRECTION('',(1.,0.,0.));
#31440=DIRECTION('center_axis',(0.,1.,0.));
#31441=DIRECTION('ref_axis',(0.,0.,1.));
#31442=DIRECTION('',(0.,0.,1.));
#31443=DIRECTION('',(1.,0.,0.));
#31444=DIRECTION('center_axis',(0.,0.,-1.));
#31445=DIRECTION('ref_axis',(0.,1.,0.));
#31446=DIRECTION('',(0.,1.,0.));
#31447=DIRECTION('center_axis',(1.,0.,0.));
#31448=DIRECTION('ref_axis',(0.,0.,-1.));
#49920=CARTESIAN_POINT('',(0.,0.,0.));
#49921=CARTESIAN_POINT('Origin',(1.5,-1.9,1.7));
#49922=CARTESIAN_POINT('',(1.56403124237433,-1.7,1.7));
#49923=CARTESIAN_POINT('',(1.43596875762567,-1.7,1.7));
#49924=CARTESIAN_POINT('',(0.75,-1.7,1.7));
#49925=CARTESIAN_POINT('Origin',(1.5,-1.9,1.7));
#49926=CARTESIAN_POINT('Origin',(1.5,-1.9,1.7));
#49927=CARTESIAN_POINT('',(1.56403124237433,-1.7,1.75));
#49928=CARTESIAN_POINT('',(1.56403124237433,-1.7,1.7));
#49929=CARTESIAN_POINT('',(1.29,-1.9,1.75));
#49930=CARTESIAN_POINT('Origin',(1.5,-1.9,1.75));
#49931=CARTESIAN_POINT('',(1.29,-1.9,2.4));
#49932=CARTESIAN_POINT('',(1.29,-1.9,1.7));
#49933=CARTESIAN_POINT('Origin',(1.5,-1.9,2.4));
#49934=CARTESIAN_POINT('',(1.43596875762567,-1.7,1.75));
#49935=CARTESIAN_POINT('Origin',(1.5,-1.9,1.75));
#49936=CARTESIAN_POINT('',(1.43596875762567,-1.7,1.7));
#49937=CARTESIAN_POINT('Origin',(-1.5,1.9,1.7));
#49938=CARTESIAN_POINT('',(-1.56403124237433,1.7,1.7));
#49939=CARTESIAN_POINT('',(-1.43596875762567,1.7,1.7));
#49940=CARTESIAN_POINT('',(-0.75,1.7,1.7));
#49941=CARTESIAN_POINT('Origin',(-1.5,1.9,1.7));
#49942=CARTESIAN_POINT('Origin',(-1.5,1.9,1.7));
#49943=CARTESIAN_POINT('',(-1.56403124237433,1.7,1.75));
#49944=CARTESIAN_POINT('',(-1.56403124237433,1.7,1.7));
#49945=CARTESIAN_POINT('',(-1.71,1.9,1.75));
#49946=CARTESIAN_POINT('Origin',(-1.5,1.9,1.75));
#49947=CARTESIAN_POINT('',(-1.71,1.9,2.4));
#49948=CARTESIAN_POINT('',(-1.71,1.9,1.7));
#49949=CARTESIAN_POINT('Origin',(-1.5,1.9,2.4));
#49950=CARTESIAN_POINT('',(-1.43596875762567,1.7,1.75));
#49951=CARTESIAN_POINT('Origin',(-1.5,1.9,1.75));
#49952=CARTESIAN_POINT('',(-1.43596875762567,1.7,1.7));
#49953=CARTESIAN_POINT('Origin',(-1.5,-1.9,1.7));
#49954=CARTESIAN_POINT('',(-1.43596875762567,-1.7,1.7));
#49955=CARTESIAN_POINT('',(-1.56403124237433,-1.7,1.7));
#49956=CARTESIAN_POINT('',(-0.75,-1.7,1.7));
#49957=CARTESIAN_POINT('Origin',(-1.5,-1.9,1.7));
#49958=CARTESIAN_POINT('Origin',(-1.5,-1.9,1.7));
#49959=CARTESIAN_POINT('',(-1.43596875762567,-1.7,1.75));
#49960=CARTESIAN_POINT('',(-1.43596875762567,-1.7,1.7));
#49961=CARTESIAN_POINT('',(-1.71,-1.9,1.75));
#49962=CARTESIAN_POINT('Origin',(-1.5,-1.9,1.75));
#49963=CARTESIAN_POINT('',(-1.71,-1.9,2.4));
#49964=CARTESIAN_POINT('',(-1.71,-1.9,1.7));
#49965=CARTESIAN_POINT('Origin',(-1.5,-1.9,2.4));
#49966=CARTESIAN_POINT('',(-1.56403124237433,-1.7,1.75));
#49967=CARTESIAN_POINT('Origin',(-1.5,-1.9,1.75));
#49968=CARTESIAN_POINT('',(-1.56403124237433,-1.7,1.7));
#49969=CARTESIAN_POINT('Origin',(1.5,1.9,1.7));
#49970=CARTESIAN_POINT('',(1.43596875762567,1.7,1.7));
#49971=CARTESIAN_POINT('',(1.56403124237433,1.7,1.7));
#49972=CARTESIAN_POINT('',(0.75,1.7,1.7));
#49973=CARTESIAN_POINT('Origin',(1.5,1.9,1.7));
#49974=CARTESIAN_POINT('Origin',(1.5,1.9,1.7));
#49975=CARTESIAN_POINT('',(1.43596875762567,1.7,1.75));
#49976=CARTESIAN_POINT('',(1.43596875762567,1.7,1.7));
#49977=CARTESIAN_POINT('',(1.29,1.9,1.75));
#49978=CARTESIAN_POINT('Origin',(1.5,1.9,1.75));
#49979=CARTESIAN_POINT('',(1.29,1.9,2.4));
#49980=CARTESIAN_POINT('',(1.29,1.9,1.7));
#49981=CARTESIAN_POINT('Origin',(1.5,1.9,2.4));
#49982=CARTESIAN_POINT('',(1.56403124237433,1.7,1.75));
#49983=CARTESIAN_POINT('Origin',(1.5,1.9,1.75));
#49984=CARTESIAN_POINT('',(1.56403124237433,1.7,1.7));
#49985=CARTESIAN_POINT('Origin',(0.,-1.7,1.75));
#49986=CARTESIAN_POINT('',(0.,-1.7,1.75));
#49987=CARTESIAN_POINT('',(-1.97,-1.7,1.75));
#49988=CARTESIAN_POINT('',(0.,-1.7,1.75));
#49989=CARTESIAN_POINT('',(-1.97,-1.7,0.43));
#49990=CARTESIAN_POINT('',(-1.97,-1.7,1.75));
#49991=CARTESIAN_POINT('',(1.97,-1.7,0.43));
#49992=CARTESIAN_POINT('',(0.,-1.7,0.43));
#49993=CARTESIAN_POINT('',(1.97,-1.7,1.75));
#49994=CARTESIAN_POINT('',(1.97,-1.7,1.75));
#49995=CARTESIAN_POINT('',(0.,-1.7,1.75));
#49996=CARTESIAN_POINT('Origin',(0.,1.7,0.43));
#49997=CARTESIAN_POINT('',(0.,1.7,1.75));
#49998=CARTESIAN_POINT('',(1.97,1.7,1.75));
#49999=CARTESIAN_POINT('',(0.,1.7,1.75));
#50000=CARTESIAN_POINT('',(1.97,1.7,0.43));
#50001=CARTESIAN_POINT('',(1.97,1.7,0.43));
#50002=CARTESIAN_POINT('',(-1.97,1.7,0.43));
#50003=CARTESIAN_POINT('',(0.,1.7,0.43));
#50004=CARTESIAN_POINT('',(-1.97,1.7,1.75));
#50005=CARTESIAN_POINT('',(-1.97,1.7,0.43));
#50006=CARTESIAN_POINT('',(0.,1.7,1.75));
#50007=CARTESIAN_POINT('Origin',(-1.97,0.,1.415));
#50008=CARTESIAN_POINT('',(-1.97,-2.35,1.75));
#50009=CARTESIAN_POINT('',(-1.97,-2.35,1.75));
#50010=CARTESIAN_POINT('',(-1.97,-2.35,2.4));
#50011=CARTESIAN_POINT('',(-1.97,-2.35,2.4));
#50012=CARTESIAN_POINT('',(-1.97,2.35,2.4));
#50013=CARTESIAN_POINT('',(-1.97,2.35,2.4));
#50014=CARTESIAN_POINT('',(-1.97,2.35,1.75));
#50015=CARTESIAN_POINT('',(-1.97,2.35,1.75));
#50016=CARTESIAN_POINT('',(-1.97,1.7,1.75));
#50017=CARTESIAN_POINT('',(-1.97,0.78,0.43));
#50018=CARTESIAN_POINT('',(-1.97,0.78,0.43));
#50019=CARTESIAN_POINT('',(-1.97,0.78,1.55));
#50020=CARTESIAN_POINT('',(-1.97,0.78,1.55));
#50021=CARTESIAN_POINT('',(-1.97,-0.78,1.55));
#50022=CARTESIAN_POINT('',(-1.97,-0.78,1.55));
#50023=CARTESIAN_POINT('',(-1.97,-0.78,0.43));
#50024=CARTESIAN_POINT('',(-1.97,-0.78,0.43));
#50025=CARTESIAN_POINT('',(-1.97,-1.7,0.43));
#50026=CARTESIAN_POINT('Origin',(0.,-2.35,1.75));
#50027=CARTESIAN_POINT('',(1.97,-2.35,1.75));
#50028=CARTESIAN_POINT('',(1.97,-2.35,1.75));
#50029=CARTESIAN_POINT('',(0.,-2.35,1.75));
#50030=CARTESIAN_POINT('Origin',(0.,-2.35,2.4));
#50031=CARTESIAN_POINT('',(1.97,-2.35,2.4));
#50032=CARTESIAN_POINT('',(1.97,-2.35,2.4));
#50033=CARTESIAN_POINT('',(0.,-2.35,2.4));
#50034=CARTESIAN_POINT('Origin',(0.,2.35,2.4));
#50035=CARTESIAN_POINT('',(1.97,2.35,2.4));
#50036=CARTESIAN_POINT('',(1.97,2.35,2.4));
#50037=CARTESIAN_POINT('',(0.,2.35,2.4));
#50038=CARTESIAN_POINT('Origin',(0.,2.35,1.75));
#50039=CARTESIAN_POINT('',(1.97,2.35,1.75));
#50040=CARTESIAN_POINT('',(1.97,2.35,1.75));
#50041=CARTESIAN_POINT('',(0.,2.35,1.75));
#50042=CARTESIAN_POINT('Origin',(0.,1.7,1.75));
#50043=CARTESIAN_POINT('',(1.97,1.7,1.75));
#50044=CARTESIAN_POINT('Origin',(0.,0.78,0.43));
#50045=CARTESIAN_POINT('',(1.97,0.78,0.43));
#50046=CARTESIAN_POINT('',(1.97,0.78,0.43));
#50047=CARTESIAN_POINT('',(0.,0.78,0.43));
#50048=CARTESIAN_POINT('Origin',(0.,0.78,1.55));
#50049=CARTESIAN_POINT('',(1.97,0.78,1.55));
#50050=CARTESIAN_POINT('',(1.97,0.78,1.55));
#50051=CARTESIAN_POINT('',(0.,0.78,1.55));
#50052=CARTESIAN_POINT('Origin',(0.,-0.78,1.55));
#50053=CARTESIAN_POINT('',(1.97,-0.78,1.55));
#50054=CARTESIAN_POINT('',(1.97,-0.78,1.55));
#50055=CARTESIAN_POINT('',(0.,-0.78,1.55));
#50056=CARTESIAN_POINT('Origin',(0.,-0.78,0.43));
#50057=CARTESIAN_POINT('',(1.97,-0.78,0.43));
#50058=CARTESIAN_POINT('',(1.97,-0.78,0.43));
#50059=CARTESIAN_POINT('',(0.,-0.78,0.43));
#50060=CARTESIAN_POINT('Origin',(0.,-1.7,0.43));
#50061=CARTESIAN_POINT('',(1.97,-1.7,0.43));
#50062=CARTESIAN_POINT('Origin',(1.97,0.,1.415));
#62866=UNCERTAINTY_MEASURE_WITH_UNIT(LENGTH_MEASURE(0.001),#62985,
'DISTANCE_ACCURACY_VALUE',
'Maximum model space distance between geometric entities at asserted c
onnectivities');
#62885=UNCERTAINTY_MEASURE_WITH_UNIT(LENGTH_MEASURE(0.001),#62985,
'DISTANCE_ACCURACY_VALUE',
'Maximum model space distance between geometric entities at asserted c
onnectivities');
#62965=(
GEOMETRIC_REPRESENTATION_CONTEXT(3)
GLOBAL_UNCERTAINTY_ASSIGNED_CONTEXT((#62866))
GLOBAL_UNIT_ASSIGNED_CONTEXT((#62985,#62987,#62988))
REPRESENTATION_CONTEXT('','3D')
);
#62984=(
GEOMETRIC_REPRESENTATION_CONTEXT(3)
GLOBAL_UNCERTAINTY_ASSIGNED_CONTEXT((#62885))
GLOBAL_UNIT_ASSIGNED_CONTEXT((#62985,#62987,#62988))
REPRESENTATION_CONTEXT('','3D')
);
#62985=(
LENGTH_UNIT()
NAMED_UNIT(*)
SI_UNIT(.CENTI.,.METRE.)
);
#62987=(
NAMED_UNIT(*)
PLANE_ANGLE_UNIT()
SI_UNIT($,.RADIAN.)
);
#62988=(
NAMED_UNIT(*)
SI_UNIT($,.STERADIAN.)
SOLID_ANGLE_UNIT()
);
#63068=SHAPE_DEFINITION_REPRESENTATION(#63256,#63428);
#63256=PRODUCT_DEFINITION_SHAPE('',$,#63527);
#63428=SHAPE_REPRESENTATION('',(#25906),#62965);
#63447=PRODUCT_DEFINITION_CONTEXT('part definition',#63743,'design');
#63527=PRODUCT_DEFINITION('Block (1)','Block (1)',#63625,#63447);
#63625=PRODUCT_DEFINITION_FORMATION('',$,#63824);
#63743=APPLICATION_CONTEXT(
'Core Data for Automotive Mechanical Design Process');
#63744=PRODUCT_CONTEXT('part definition',#63743,'mechanical');
#63824=PRODUCT('Block (1)','Block (1)','Block (1)',(#63744));
#63885=COLOUR_RGB('Dark Blue',0.08,0.2,0.34);
#63886=FILL_AREA_STYLE_COLOUR('',#63885);
#63887=FILL_AREA_STYLE('',(#63886));
#63888=SURFACE_STYLE_FILL_AREA(#63887);
#63889=SURFACE_SIDE_STYLE('',(#63888));
#63890=SURFACE_STYLE_USAGE(.BOTH.,#63889);
#63891=PRESENTATION_STYLE_ASSIGNMENT((#63890));
ENDSEC;
END-ISO-10303-21;
